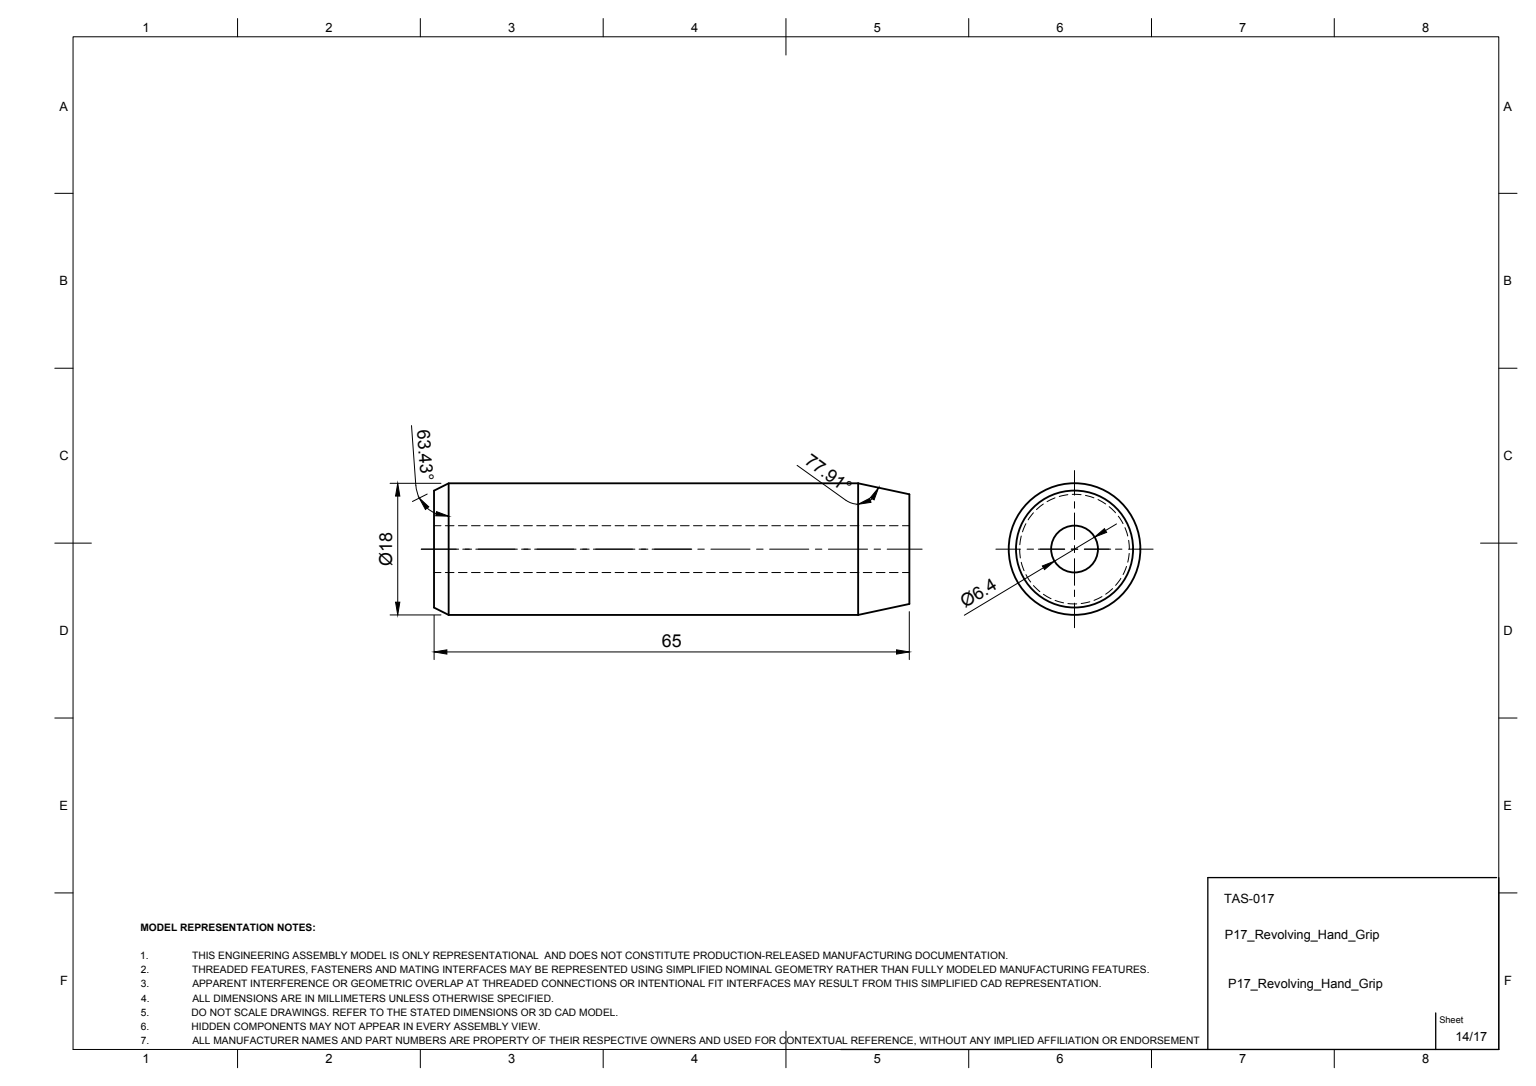
ISO-10303-21;
HEADER;
/* Generated by software containing ST-Developer
 * from STEP Tools, Inc. (www.steptools.com) 
 */

FILE_DESCRIPTION(
/* description */ ('STEP AP203'),
/* implementation_level */ '2;1');

FILE_NAME(
/* name */ 'P17_Revolving_Hand_Grip.step',
/* time_stamp */ '2026-11-15T15:04:01-08:00',
/* author */ (''),
/* organization */ (''),
/* preprocessor_version */ 'ST-DEVELOPER v20.2',
/* originating_system */ 'Autodesk Translation Framework v15.17.0.0',
/* authorisation */ '');

FILE_SCHEMA (('AUTOMOTIVE_DESIGN { 1 0 10303 214 3 1 1 }'));
ENDSEC;

DATA;
#10=MECHANICAL_DESIGN_GEOMETRIC_PRESENTATION_REPRESENTATION('',(#300),#16598);
#187=CONICAL_SURFACE('',#10802,7.5,0.211093333222747);
#188=CONICAL_SURFACE('',#10808,9.,0.463647609000806);
#222=SHAPE_REPRESENTATION_RELATIONSHIP('SRR','None',#16716,#246);
#246=ADVANCED_BREP_SHAPE_REPRESENTATION('',(#270),#16592);
#270=MANIFOLD_SOLID_BREP('Body1',#9805);
#300=STYLED_ITEM('',(#16827),#270);
#419=FACE_BOUND('',#2077,.T.);
#420=FACE_BOUND('',#2079,.T.);
#869=PLANE('',#10813);
#870=PLANE('',#10814);
#1408=FACE_OUTER_BOUND('',#2072,.T.);
#1409=FACE_OUTER_BOUND('',#2073,.T.);
#1410=FACE_OUTER_BOUND('',#2074,.T.);
#1411=FACE_OUTER_BOUND('',#2075,.T.);
#1412=FACE_OUTER_BOUND('',#2076,.T.);
#1413=FACE_OUTER_BOUND('',#2078,.T.);
#2072=EDGE_LOOP('',(#8955,#8956,#8957,#8958));
#2073=EDGE_LOOP('',(#8959,#8960,#8961,#8962,#8963));
#2074=EDGE_LOOP('',(#8964,#8965,#8966,#8967,#8968));
#2075=EDGE_LOOP('',(#8969,#8970,#8971,#8972));
#2076=EDGE_LOOP('',(#8973));
#2077=EDGE_LOOP('',(#8974));
#2078=EDGE_LOOP('',(#8975));
#2079=EDGE_LOOP('',(#8976));
#3100=LINE('',#16270,#4148);
#3101=LINE('',#16277,#4149);
#3102=LINE('',#16280,#4150);
#3103=LINE('',#16286,#4151);
#4148=VECTOR('',#13348,7.5);
#4149=VECTOR('',#13357,9.);
#4150=VECTOR('',#13360,9.);
#4151=VECTOR('',#13367,3.2);
#4432=CIRCLE('',#10803,9.);
#4433=CIRCLE('',#10804,7.5);
#4434=CIRCLE('',#10806,9.);
#4435=CIRCLE('',#10807,9.);
#4436=CIRCLE('',#10809,8.);
#4437=CIRCLE('',#10811,3.2);
#4438=CIRCLE('',#10812,3.2);
#5240=VERTEX_POINT('',#16267);
#5241=VERTEX_POINT('',#16269);
#5242=VERTEX_POINT('',#16273);
#5243=VERTEX_POINT('',#16274);
#5244=VERTEX_POINT('',#16279);
#5245=VERTEX_POINT('',#16283);
#5246=VERTEX_POINT('',#16285);
#6490=EDGE_CURVE('',#5240,#5240,#4432,.T.);
#6491=EDGE_CURVE('',#5240,#5241,#3100,.T.);
#6492=EDGE_CURVE('',#5241,#5241,#4433,.T.);
#6493=EDGE_CURVE('',#5242,#5243,#4434,.T.);
#6494=EDGE_CURVE('',#5243,#5242,#4435,.T.);
#6495=EDGE_CURVE('',#5243,#5240,#3101,.T.);
#6496=EDGE_CURVE('',#5242,#5244,#3102,.T.);
#6497=EDGE_CURVE('',#5244,#5244,#4436,.T.);
#6498=EDGE_CURVE('',#5245,#5245,#4437,.T.);
#6499=EDGE_CURVE('',#5245,#5246,#3103,.T.);
#6500=EDGE_CURVE('',#5246,#5246,#4438,.T.);
#8955=ORIENTED_EDGE('',*,*,#6490,.F.);
#8956=ORIENTED_EDGE('',*,*,#6491,.T.);
#8957=ORIENTED_EDGE('',*,*,#6492,.T.);
#8958=ORIENTED_EDGE('',*,*,#6491,.F.);
#8959=ORIENTED_EDGE('',*,*,#6493,.F.);
#8960=ORIENTED_EDGE('',*,*,#6494,.F.);
#8961=ORIENTED_EDGE('',*,*,#6495,.T.);
#8962=ORIENTED_EDGE('',*,*,#6490,.T.);
#8963=ORIENTED_EDGE('',*,*,#6495,.F.);
#8964=ORIENTED_EDGE('',*,*,#6493,.T.);
#8965=ORIENTED_EDGE('',*,*,#6494,.T.);
#8966=ORIENTED_EDGE('',*,*,#6496,.T.);
#8967=ORIENTED_EDGE('',*,*,#6497,.F.);
#8968=ORIENTED_EDGE('',*,*,#6496,.F.);
#8969=ORIENTED_EDGE('',*,*,#6498,.F.);
#8970=ORIENTED_EDGE('',*,*,#6499,.T.);
#8971=ORIENTED_EDGE('',*,*,#6500,.T.);
#8972=ORIENTED_EDGE('',*,*,#6499,.F.);
#8973=ORIENTED_EDGE('',*,*,#6497,.T.);
#8974=ORIENTED_EDGE('',*,*,#6500,.F.);
#8975=ORIENTED_EDGE('',*,*,#6492,.F.);
#8976=ORIENTED_EDGE('',*,*,#6498,.T.);
#9226=CYLINDRICAL_SURFACE('',#10805,9.);
#9227=CYLINDRICAL_SURFACE('',#10810,3.2);
#9733=ADVANCED_FACE('',(#1408),#187,.T.);
#9734=ADVANCED_FACE('',(#1409),#9226,.T.);
#9735=ADVANCED_FACE('',(#1410),#188,.T.);
#9736=ADVANCED_FACE('',(#1411),#9227,.F.);
#9737=ADVANCED_FACE('',(#1412,#419),#869,.F.);
#9738=ADVANCED_FACE('',(#1413,#420),#870,.F.);
#9805=CLOSED_SHELL('',(#9733,#9734,#9735,#9736,#9737,#9738));
#10801=AXIS2_PLACEMENT_3D('',#16265,#13342,#13343);
#10802=AXIS2_PLACEMENT_3D('',#16266,#13344,#13345);
#10803=AXIS2_PLACEMENT_3D('',#16268,#13346,#13347);
#10804=AXIS2_PLACEMENT_3D('',#16271,#13349,#13350);
#10805=AXIS2_PLACEMENT_3D('',#16272,#13351,#13352);
#10806=AXIS2_PLACEMENT_3D('',#16275,#13353,#13354);
#10807=AXIS2_PLACEMENT_3D('',#16276,#13355,#13356);
#10808=AXIS2_PLACEMENT_3D('',#16278,#13358,#13359);
#10809=AXIS2_PLACEMENT_3D('',#16281,#13361,#13362);
#10810=AXIS2_PLACEMENT_3D('',#16282,#13363,#13364);
#10811=AXIS2_PLACEMENT_3D('',#16284,#13365,#13366);
#10812=AXIS2_PLACEMENT_3D('',#16287,#13368,#13369);
#10813=AXIS2_PLACEMENT_3D('',#16288,#13370,#13371);
#10814=AXIS2_PLACEMENT_3D('',#16289,#13372,#13373);
#13342=DIRECTION('axis',(0.,0.,1.));
#13343=DIRECTION('refdir',(1.,0.,0.));
#13344=DIRECTION('center_axis',(0.,0.,-1.));
#13345=DIRECTION('ref_axis',(-1.,0.,0.));
#13346=DIRECTION('center_axis',(0.,0.,-1.));
#13347=DIRECTION('ref_axis',(-1.,0.,0.));
#13348=DIRECTION('',(-0.209529088730874,2.56599127842526E-17,0.977802414077409));
#13349=DIRECTION('center_axis',(0.,0.,-1.));
#13350=DIRECTION('ref_axis',(-1.,0.,0.));
#13351=DIRECTION('center_axis',(0.,0.,-1.));
#13352=DIRECTION('ref_axis',(-1.,0.,0.));
#13353=DIRECTION('center_axis',(0.,0.,-1.));
#13354=DIRECTION('ref_axis',(-1.,0.,0.));
#13355=DIRECTION('center_axis',(0.,0.,-1.));
#13356=DIRECTION('ref_axis',(-1.,0.,0.));
#13357=DIRECTION('',(0.,0.,1.));
#13358=DIRECTION('center_axis',(0.,0.,1.));
#13359=DIRECTION('ref_axis',(1.,0.,0.));
#13360=DIRECTION('',(0.447213595499958,5.47678698264203E-17,-0.894427190999916));
#13361=DIRECTION('center_axis',(0.,0.,-1.));
#13362=DIRECTION('ref_axis',(-1.,0.,0.));
#13363=DIRECTION('center_axis',(0.,0.,-1.));
#13364=DIRECTION('ref_axis',(-1.,0.,0.));
#13365=DIRECTION('center_axis',(0.,0.,-1.));
#13366=DIRECTION('ref_axis',(-1.,0.,0.));
#13367=DIRECTION('',(0.,0.,-1.));
#13368=DIRECTION('center_axis',(0.,0.,-1.));
#13369=DIRECTION('ref_axis',(-1.,0.,0.));
#13370=DIRECTION('center_axis',(0.,0.,1.));
#13371=DIRECTION('ref_axis',(1.,0.,0.));
#13372=DIRECTION('center_axis',(0.,0.,-1.));
#13373=DIRECTION('ref_axis',(-1.,0.,0.));
#16265=CARTESIAN_POINT('',(0.,0.,0.));
#16266=CARTESIAN_POINT('Origin',(0.,0.,65.));
#16267=CARTESIAN_POINT('',(9.,-1.10218211923262E-15,58.));
#16268=CARTESIAN_POINT('Origin',(0.,0.,58.));
#16269=CARTESIAN_POINT('',(7.5,-9.18485099360515E-16,65.));
#16270=CARTESIAN_POINT('',(7.5,-9.18485099360515E-16,65.));
#16271=CARTESIAN_POINT('Origin',(0.,0.,65.));
#16272=CARTESIAN_POINT('Origin',(0.,0.,-5.));
#16273=CARTESIAN_POINT('',(-9.,1.10218211923262E-15,2.));
#16274=CARTESIAN_POINT('',(9.,-1.10218211923262E-15,2.));
#16275=CARTESIAN_POINT('Origin',(0.,0.,2.));
#16276=CARTESIAN_POINT('Origin',(0.,0.,2.));
#16277=CARTESIAN_POINT('',(9.,-1.10218211923262E-15,-5.));
#16278=CARTESIAN_POINT('Origin',(0.,0.,2.));
#16279=CARTESIAN_POINT('',(-8.,-9.79717439317883E-16,-5.55111512312578E-16));
#16280=CARTESIAN_POINT('',(-9.,-1.10218211923262E-15,2.));
#16281=CARTESIAN_POINT('Origin',(0.,0.,0.));
#16282=CARTESIAN_POINT('Origin',(0.,0.,-5.));
#16283=CARTESIAN_POINT('',(3.2,-3.91886975727153E-16,65.));
#16284=CARTESIAN_POINT('Origin',(0.,0.,65.));
#16285=CARTESIAN_POINT('',(3.2,-3.91886975727153E-16,0.));
#16286=CARTESIAN_POINT('',(3.2,-3.91886975727153E-16,-5.));
#16287=CARTESIAN_POINT('Origin',(0.,0.,0.));
#16288=CARTESIAN_POINT('Origin',(3.2,0.,0.));
#16289=CARTESIAN_POINT('Origin',(7.5,0.,65.));
#16566=UNCERTAINTY_MEASURE_WITH_UNIT(LENGTH_MEASURE(0.01),#16599,
'DISTANCE_ACCURACY_VALUE',
'Maximum model space distance between geometric entities at asserted c
onnectivities');
#16572=UNCERTAINTY_MEASURE_WITH_UNIT(LENGTH_MEASURE(0.01),#16599,
'DISTANCE_ACCURACY_VALUE',
'Maximum model space distance between geometric entities at asserted c
onnectivities');
#16592=(
GEOMETRIC_REPRESENTATION_CONTEXT(3)
GLOBAL_UNCERTAINTY_ASSIGNED_CONTEXT((#16566))
GLOBAL_UNIT_ASSIGNED_CONTEXT((#16599,#16601,#16602))
REPRESENTATION_CONTEXT('','3D')
);
#16598=(
GEOMETRIC_REPRESENTATION_CONTEXT(3)
GLOBAL_UNCERTAINTY_ASSIGNED_CONTEXT((#16572))
GLOBAL_UNIT_ASSIGNED_CONTEXT((#16599,#16601,#16602))
REPRESENTATION_CONTEXT('','3D')
);
#16599=(
LENGTH_UNIT()
NAMED_UNIT(*)
SI_UNIT(.MILLI.,.METRE.)
);
#16601=(
NAMED_UNIT(*)
PLANE_ANGLE_UNIT()
SI_UNIT($,.RADIAN.)
);
#16602=(
NAMED_UNIT(*)
SI_UNIT($,.STERADIAN.)
SOLID_ANGLE_UNIT()
);
#16622=SHAPE_DEFINITION_REPRESENTATION(#16647,#16716);
#16647=PRODUCT_DEFINITION_SHAPE('',$,#16742);
#16716=SHAPE_REPRESENTATION('',(#10801),#16592);
#16722=PRODUCT_DEFINITION_CONTEXT('part definition',#16799,'design');
#16742=PRODUCT_DEFINITION('P17_Revolving_Hand_Grip',
'P17_Revolving_Hand_Grip',#16767,#16722);
#16767=PRODUCT_DEFINITION_FORMATION('',$,#16820);
#16799=APPLICATION_CONTEXT(
'Core Data for Automotive Mechanical Design Process');
#16800=PRODUCT_CONTEXT('part definition',#16799,'mechanical');
#16820=PRODUCT('P17_Revolving_Hand_Grip','P17_Revolving_Hand_Grip',$,(#16800));
#16827=PRESENTATION_STYLE_ASSIGNMENT((#16836));
#16836=SURFACE_STYLE_USAGE(.BOTH.,#16845);
#16845=SURFACE_SIDE_STYLE('',(#16854));
#16854=SURFACE_STYLE_FILL_AREA(#16863);
#16863=FILL_AREA_STYLE('Gray',(#16872));
#16872=FILL_AREA_STYLE_COLOUR('Gray',#16881);
#16881=COLOUR_RGB('Gray',0.501960784313725,0.501960784313725,0.501960784313725);
ENDSEC;
END-ISO-10303-21;
